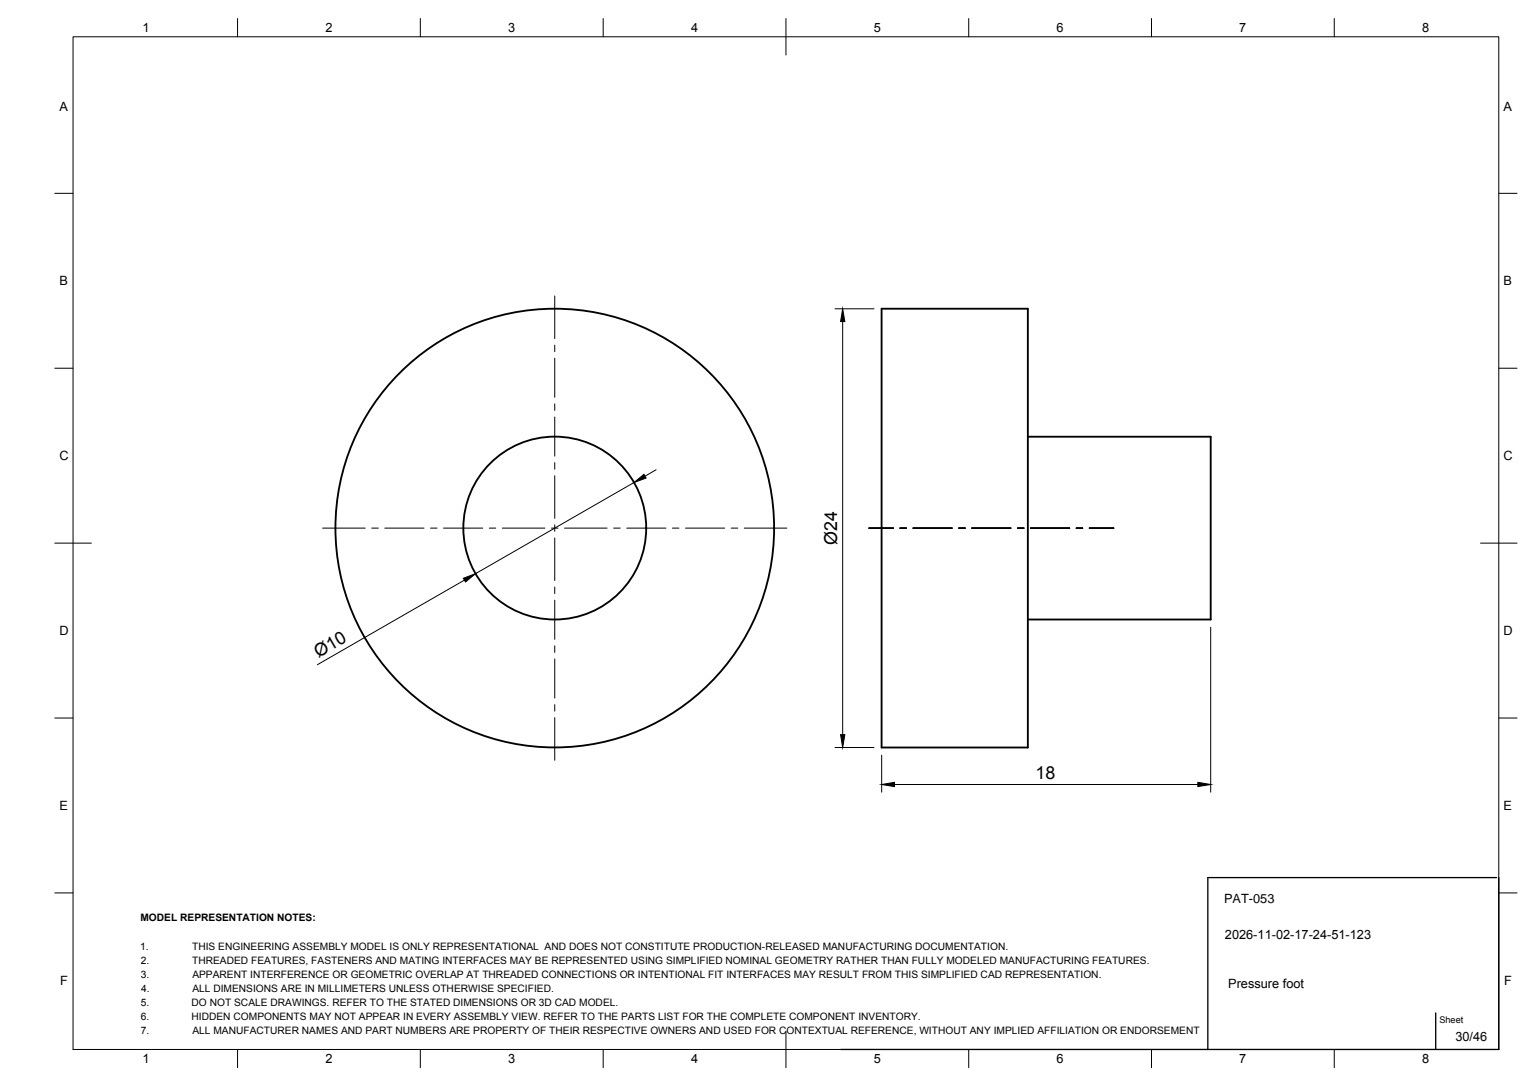
ISO-10303-21;
HEADER;
/* Generated by software containing ST-Developer
 * from STEP Tools, Inc. (www.steptools.com) 
 */

FILE_DESCRIPTION(
/* description */ ('Hand-operated arbor press'),
/* implementation_level */ '2;1');

FILE_NAME(
/* name */ 'Pressure foot.step',
/* time_stamp */ '2026-10-28T03:25:25-07:00',
/* author */ (''),
/* organization */ (''),
/* preprocessor_version */ 'ST-DEVELOPER v20.2',
/* originating_system */ 'Autodesk Translation Framework v15.17.0.0',
/* authorisation */ '');

FILE_SCHEMA (('AUTOMOTIVE_DESIGN { 1 0 10303 214 3 1 1 }'));
ENDSEC;

DATA;
#10=MECHANICAL_DESIGN_GEOMETRIC_PRESENTATION_REPRESENTATION('',(#616),#32751);
#525=SHAPE_REPRESENTATION_RELATIONSHIP('SRR','None',#32956,#567);
#567=ADVANCED_BREP_SHAPE_REPRESENTATION('',(#663),#32730);
#616=STYLED_ITEM('',(#33256),#663);
#663=MANIFOLD_SOLID_BREP('Body1',#12515);
#813=FACE_BOUND('',#2566,.T.);
#1174=PLANE('',#13752);
#1175=PLANE('',#13756);
#1176=PLANE('',#13757);
#1748=FACE_OUTER_BOUND('',#2562,.T.);
#1749=FACE_OUTER_BOUND('',#2563,.T.);
#1750=FACE_OUTER_BOUND('',#2564,.T.);
#1751=FACE_OUTER_BOUND('',#2565,.T.);
#1752=FACE_OUTER_BOUND('',#2567,.T.);
#2562=EDGE_LOOP('',(#10614,#10615,#10616,#10617));
#2563=EDGE_LOOP('',(#10618));
#2564=EDGE_LOOP('',(#10619,#10620,#10621,#10622));
#2565=EDGE_LOOP('',(#10623));
#2566=EDGE_LOOP('',(#10624));
#2567=EDGE_LOOP('',(#10625));
#3693=LINE('',#20338,#4864);
#3694=LINE('',#20345,#4865);
#4864=VECTOR('',#16528,0.5);
#4865=VECTOR('',#16537,1.2);
#5428=CIRCLE('',#13750,0.5);
#5429=CIRCLE('',#13751,0.5);
#5430=CIRCLE('',#13754,1.2);
#5431=CIRCLE('',#13755,1.2);
#6325=VERTEX_POINT('',#20335);
#6326=VERTEX_POINT('',#20337);
#6327=VERTEX_POINT('',#20342);
#6328=VERTEX_POINT('',#20344);
#7810=EDGE_CURVE('',#6325,#6325,#5428,.T.);
#7811=EDGE_CURVE('',#6325,#6326,#3693,.T.);
#7812=EDGE_CURVE('',#6326,#6326,#5429,.T.);
#7813=EDGE_CURVE('',#6327,#6327,#5430,.T.);
#7814=EDGE_CURVE('',#6327,#6328,#3694,.T.);
#7815=EDGE_CURVE('',#6328,#6328,#5431,.T.);
#10614=ORIENTED_EDGE('',*,*,#7810,.F.);
#10615=ORIENTED_EDGE('',*,*,#7811,.T.);
#10616=ORIENTED_EDGE('',*,*,#7812,.F.);
#10617=ORIENTED_EDGE('',*,*,#7811,.F.);
#10618=ORIENTED_EDGE('',*,*,#7810,.T.);
#10619=ORIENTED_EDGE('',*,*,#7813,.F.);
#10620=ORIENTED_EDGE('',*,*,#7814,.T.);
#10621=ORIENTED_EDGE('',*,*,#7815,.T.);
#10622=ORIENTED_EDGE('',*,*,#7814,.F.);
#10623=ORIENTED_EDGE('',*,*,#7813,.T.);
#10624=ORIENTED_EDGE('',*,*,#7812,.T.);
#10625=ORIENTED_EDGE('',*,*,#7815,.F.);
#11745=CYLINDRICAL_SURFACE('',#13749,0.5);
#11746=CYLINDRICAL_SURFACE('',#13753,1.2);
#12257=ADVANCED_FACE('',(#1748),#11745,.T.);
#12258=ADVANCED_FACE('',(#1749),#1174,.T.);
#12259=ADVANCED_FACE('',(#1750),#11746,.T.);
#12260=ADVANCED_FACE('',(#1751,#813),#1175,.T.);
#12261=ADVANCED_FACE('',(#1752),#1176,.F.);
#12515=CLOSED_SHELL('',(#12257,#12258,#12259,#12260,#12261));
#13748=AXIS2_PLACEMENT_3D('',#20333,#16522,#16523);
#13749=AXIS2_PLACEMENT_3D('',#20334,#16524,#16525);
#13750=AXIS2_PLACEMENT_3D('',#20336,#16526,#16527);
#13751=AXIS2_PLACEMENT_3D('',#20339,#16529,#16530);
#13752=AXIS2_PLACEMENT_3D('',#20340,#16531,#16532);
#13753=AXIS2_PLACEMENT_3D('',#20341,#16533,#16534);
#13754=AXIS2_PLACEMENT_3D('',#20343,#16535,#16536);
#13755=AXIS2_PLACEMENT_3D('',#20346,#16538,#16539);
#13756=AXIS2_PLACEMENT_3D('',#20347,#16540,#16541);
#13757=AXIS2_PLACEMENT_3D('',#20348,#16542,#16543);
#16522=DIRECTION('axis',(0.,0.,1.));
#16523=DIRECTION('refdir',(1.,0.,0.));
#16524=DIRECTION('center_axis',(0.,0.,1.));
#16525=DIRECTION('ref_axis',(1.,0.,0.));
#16526=DIRECTION('center_axis',(0.,0.,1.));
#16527=DIRECTION('ref_axis',(1.,0.,0.));
#16528=DIRECTION('',(0.,0.,-1.));
#16529=DIRECTION('center_axis',(0.,0.,-1.));
#16530=DIRECTION('ref_axis',(1.,0.,0.));
#16531=DIRECTION('center_axis',(0.,0.,1.));
#16532=DIRECTION('ref_axis',(1.,0.,0.));
#16533=DIRECTION('center_axis',(0.,0.,1.));
#16534=DIRECTION('ref_axis',(1.,0.,0.));
#16535=DIRECTION('center_axis',(0.,0.,1.));
#16536=DIRECTION('ref_axis',(1.,0.,0.));
#16537=DIRECTION('',(0.,0.,-1.));
#16538=DIRECTION('center_axis',(0.,0.,1.));
#16539=DIRECTION('ref_axis',(1.,0.,0.));
#16540=DIRECTION('center_axis',(0.,0.,1.));
#16541=DIRECTION('ref_axis',(1.,0.,0.));
#16542=DIRECTION('center_axis',(0.,0.,1.));
#16543=DIRECTION('ref_axis',(1.,0.,0.));
#20333=CARTESIAN_POINT('',(0.,0.,0.));
#20334=CARTESIAN_POINT('Origin',(1.,0.,10.8));
#20335=CARTESIAN_POINT('',(0.5,-6.12323399573677E-17,11.8));
#20336=CARTESIAN_POINT('Origin',(1.,0.,11.8));
#20337=CARTESIAN_POINT('',(0.5,-6.12323399573677E-17,10.8));
#20338=CARTESIAN_POINT('',(0.5,-6.12323399573677E-17,10.8));
#20339=CARTESIAN_POINT('Origin',(1.,0.,10.8));
#20340=CARTESIAN_POINT('Origin',(1.,0.,11.8));
#20341=CARTESIAN_POINT('Origin',(1.,0.,10.));
#20342=CARTESIAN_POINT('',(-0.2,-1.46957615897682E-16,10.8));
#20343=CARTESIAN_POINT('Origin',(1.,0.,10.8));
#20344=CARTESIAN_POINT('',(-0.2,-1.46957615897682E-16,10.));
#20345=CARTESIAN_POINT('',(-0.2,-1.46957615897682E-16,10.));
#20346=CARTESIAN_POINT('Origin',(1.,0.,10.));
#20347=CARTESIAN_POINT('Origin',(1.,0.,10.8));
#20348=CARTESIAN_POINT('Origin',(1.,0.,10.));
#32681=UNCERTAINTY_MEASURE_WITH_UNIT(LENGTH_MEASURE(0.001),#32752,
'DISTANCE_ACCURACY_VALUE',
'Maximum model space distance between geometric entities at asserted c
onnectivities');
#32702=UNCERTAINTY_MEASURE_WITH_UNIT(LENGTH_MEASURE(0.001),#32752,
'DISTANCE_ACCURACY_VALUE',
'Maximum model space distance between geometric entities at asserted c
onnectivities');
#32730=(
GEOMETRIC_REPRESENTATION_CONTEXT(3)
GLOBAL_UNCERTAINTY_ASSIGNED_CONTEXT((#32681))
GLOBAL_UNIT_ASSIGNED_CONTEXT((#32752,#32754,#32755))
REPRESENTATION_CONTEXT('','3D')
);
#32751=(
GEOMETRIC_REPRESENTATION_CONTEXT(3)
GLOBAL_UNCERTAINTY_ASSIGNED_CONTEXT((#32702))
GLOBAL_UNIT_ASSIGNED_CONTEXT((#32752,#32754,#32755))
REPRESENTATION_CONTEXT('','3D')
);
#32752=(
LENGTH_UNIT()
NAMED_UNIT(*)
SI_UNIT(.CENTI.,.METRE.)
);
#32754=(
NAMED_UNIT(*)
PLANE_ANGLE_UNIT()
SI_UNIT($,.RADIAN.)
);
#32755=(
NAMED_UNIT(*)
SI_UNIT($,.STERADIAN.)
SOLID_ANGLE_UNIT()
);
#32783=SHAPE_DEFINITION_REPRESENTATION(#32836,#32956);
#32836=PRODUCT_DEFINITION_SHAPE('',$,#33005);
#32956=SHAPE_REPRESENTATION('',(#13748),#32730);
#32977=PRODUCT_DEFINITION_CONTEXT('part definition',#33123,'design');
#33005=PRODUCT_DEFINITION('Pressure foot','Pressure foot',#33053,#32977);
#33053=PRODUCT_DEFINITION_FORMATION('',$,#33152);
#33123=APPLICATION_CONTEXT(
'Core Data for Automotive Mechanical Design Process');
#33124=PRODUCT_CONTEXT('part definition',#33123,'mechanical');
#33152=PRODUCT('Pressure foot','Pressure foot','Pressure foot',(#33124));
#33250=COLOUR_RGB('Off White',0.89,0.88,0.83);
#33251=FILL_AREA_STYLE_COLOUR('',#33250);
#33252=FILL_AREA_STYLE('',(#33251));
#33253=SURFACE_STYLE_FILL_AREA(#33252);
#33254=SURFACE_SIDE_STYLE('',(#33253));
#33255=SURFACE_STYLE_USAGE(.BOTH.,#33254);
#33256=PRESENTATION_STYLE_ASSIGNMENT((#33255));
ENDSEC;
END-ISO-10303-21;
